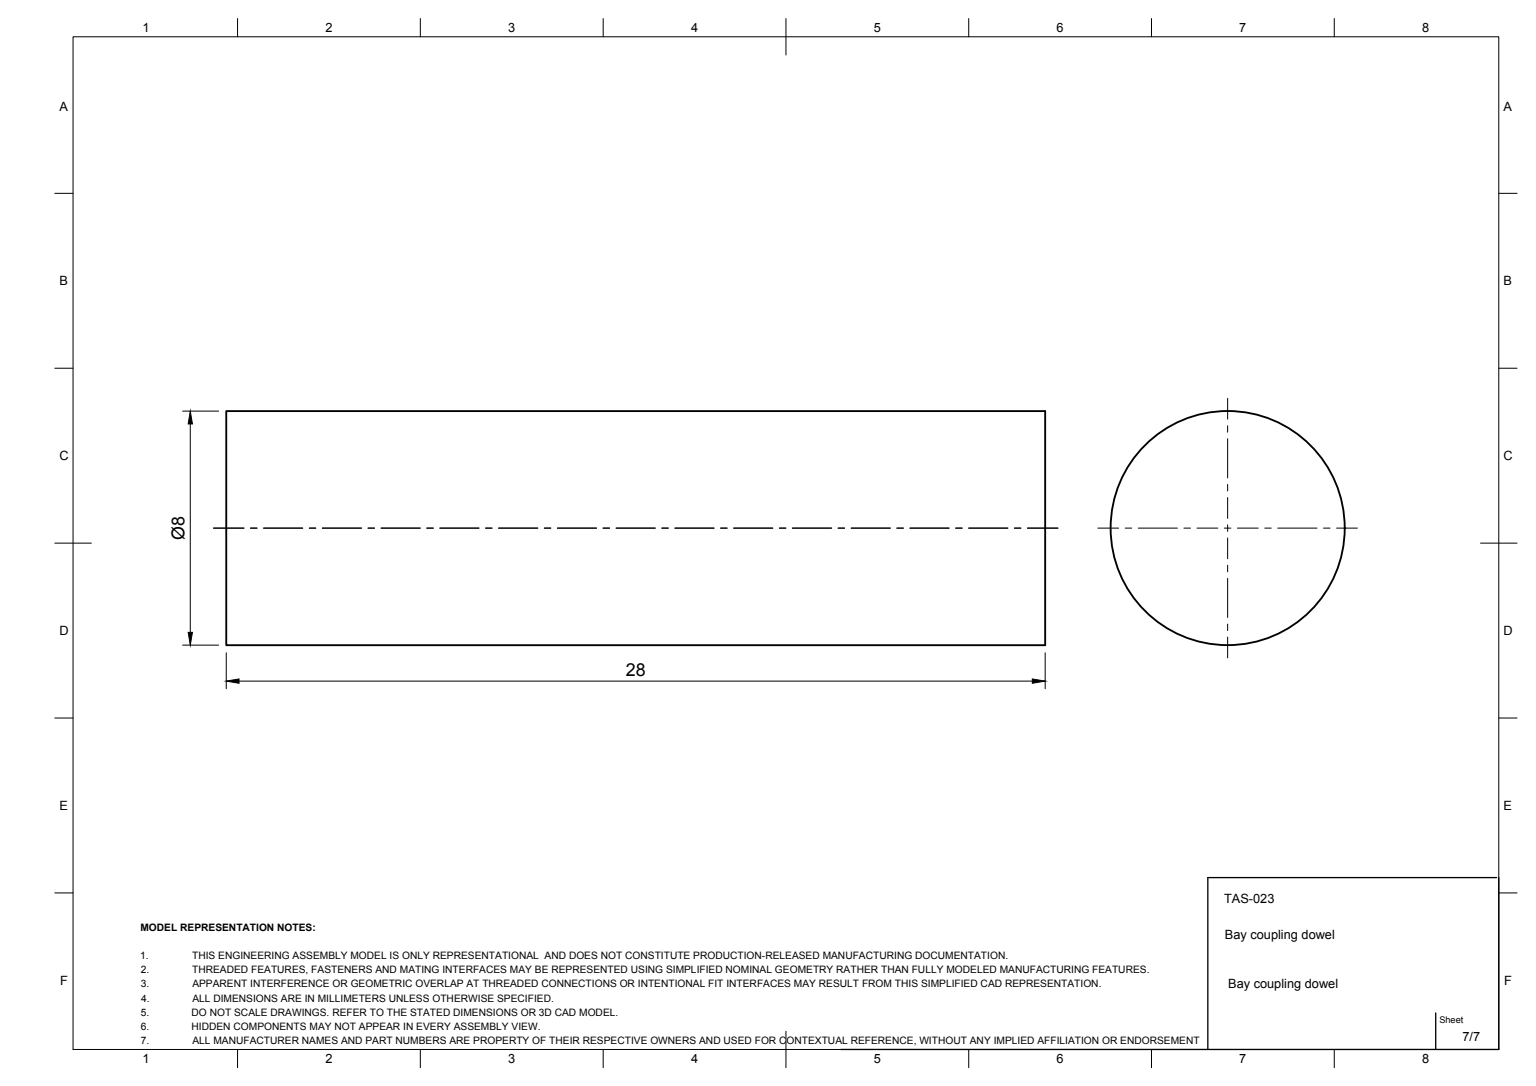
ISO-10303-21;
HEADER;
/* Generated by software containing ST-Developer
 * from STEP Tools, Inc. (www.steptools.com) 
 */

FILE_DESCRIPTION(
/* description */ (''),
/* implementation_level */ '2;1');

FILE_NAME(
/* name */ 'Bay coupling dowel.step',
/* time_stamp */ '2026-11-15T17:51:54-08:00',
/* author */ (''),
/* organization */ (''),
/* preprocessor_version */ 'ST-DEVELOPER v20.2',
/* originating_system */ 'Autodesk Translation Framework v15.17.0.0',
/* authorisation */ '');

FILE_SCHEMA (('AUTOMOTIVE_DESIGN { 1 0 10303 214 3 1 1 }'));
ENDSEC;

DATA;
#10=MECHANICAL_DESIGN_GEOMETRIC_PRESENTATION_REPRESENTATION('',(#121),#2860);
#111=SHAPE_REPRESENTATION_RELATIONSHIP('SRR','None',#2906,#116);
#116=ADVANCED_BREP_SHAPE_REPRESENTATION('',(#126),#2859);
#121=STYLED_ITEM('',(#2940),#126);
#126=MANIFOLD_SOLID_BREP('Body1',#1718);
#211=PLANE('',#1876);
#212=PLANE('',#1877);
#297=FACE_OUTER_BOUND('',#388,.T.);
#298=FACE_OUTER_BOUND('',#389,.T.);
#299=FACE_OUTER_BOUND('',#390,.T.);
#388=EDGE_LOOP('',(#1616,#1617,#1618,#1619));
#389=EDGE_LOOP('',(#1620));
#390=EDGE_LOOP('',(#1621));
#599=LINE('',#2819,#808);
#808=VECTOR('',#2310,0.4);
#817=CIRCLE('',#1874,0.4);
#818=CIRCLE('',#1875,0.4);
#963=VERTEX_POINT('',#2816);
#964=VERTEX_POINT('',#2818);
#1181=EDGE_CURVE('',#963,#963,#817,.T.);
#1182=EDGE_CURVE('',#963,#964,#599,.T.);
#1183=EDGE_CURVE('',#964,#964,#818,.T.);
#1616=ORIENTED_EDGE('',*,*,#1181,.F.);
#1617=ORIENTED_EDGE('',*,*,#1182,.T.);
#1618=ORIENTED_EDGE('',*,*,#1183,.T.);
#1619=ORIENTED_EDGE('',*,*,#1182,.F.);
#1620=ORIENTED_EDGE('',*,*,#1181,.T.);
#1621=ORIENTED_EDGE('',*,*,#1183,.F.);
#1626=CYLINDRICAL_SURFACE('',#1873,0.4);
#1711=ADVANCED_FACE('',(#297),#1626,.T.);
#1712=ADVANCED_FACE('',(#298),#211,.T.);
#1713=ADVANCED_FACE('',(#299),#212,.F.);
#1718=CLOSED_SHELL('',(#1711,#1712,#1713));
#1872=AXIS2_PLACEMENT_3D('',#2814,#2304,#2305);
#1873=AXIS2_PLACEMENT_3D('',#2815,#2306,#2307);
#1874=AXIS2_PLACEMENT_3D('',#2817,#2308,#2309);
#1875=AXIS2_PLACEMENT_3D('',#2820,#2311,#2312);
#1876=AXIS2_PLACEMENT_3D('',#2821,#2313,#2314);
#1877=AXIS2_PLACEMENT_3D('',#2822,#2315,#2316);
#2304=DIRECTION('axis',(0.,0.,1.));
#2305=DIRECTION('refdir',(1.,0.,0.));
#2306=DIRECTION('center_axis',(0.,0.,1.));
#2307=DIRECTION('ref_axis',(1.,0.,0.));
#2308=DIRECTION('center_axis',(0.,0.,1.));
#2309=DIRECTION('ref_axis',(1.,0.,0.));
#2310=DIRECTION('',(0.,0.,-1.));
#2311=DIRECTION('center_axis',(0.,0.,1.));
#2312=DIRECTION('ref_axis',(1.,0.,0.));
#2313=DIRECTION('center_axis',(0.,0.,1.));
#2314=DIRECTION('ref_axis',(1.,0.,0.));
#2315=DIRECTION('center_axis',(0.,0.,1.));
#2316=DIRECTION('ref_axis',(1.,0.,0.));
#2814=CARTESIAN_POINT('',(0.,0.,0.));
#2815=CARTESIAN_POINT('Origin',(0.,0.,0.));
#2816=CARTESIAN_POINT('',(-0.4,-4.89858719658941E-17,2.8));
#2817=CARTESIAN_POINT('Origin',(0.,0.,2.8));
#2818=CARTESIAN_POINT('',(-0.4,-4.89858719658941E-17,0.));
#2819=CARTESIAN_POINT('',(-0.4,-4.89858719658941E-17,0.));
#2820=CARTESIAN_POINT('Origin',(0.,0.,0.));
#2821=CARTESIAN_POINT('Origin',(0.,0.,2.8));
#2822=CARTESIAN_POINT('Origin',(0.,0.,0.));
#2852=UNCERTAINTY_MEASURE_WITH_UNIT(LENGTH_MEASURE(0.001),#2861,
'DISTANCE_ACCURACY_VALUE',
'Maximum model space distance between geometric entities at asserted c
onnectivities');
#2853=UNCERTAINTY_MEASURE_WITH_UNIT(LENGTH_MEASURE(0.001),#2861,
'DISTANCE_ACCURACY_VALUE',
'Maximum model space distance between geometric entities at asserted c
onnectivities');
#2859=(
GEOMETRIC_REPRESENTATION_CONTEXT(3)
GLOBAL_UNCERTAINTY_ASSIGNED_CONTEXT((#2852))
GLOBAL_UNIT_ASSIGNED_CONTEXT((#2861,#2863,#2864))
REPRESENTATION_CONTEXT('','3D')
);
#2860=(
GEOMETRIC_REPRESENTATION_CONTEXT(3)
GLOBAL_UNCERTAINTY_ASSIGNED_CONTEXT((#2853))
GLOBAL_UNIT_ASSIGNED_CONTEXT((#2861,#2863,#2864))
REPRESENTATION_CONTEXT('','3D')
);
#2861=(
LENGTH_UNIT()
NAMED_UNIT(*)
SI_UNIT(.CENTI.,.METRE.)
);
#2863=(
NAMED_UNIT(*)
PLANE_ANGLE_UNIT()
SI_UNIT($,.RADIAN.)
);
#2864=(
NAMED_UNIT(*)
SI_UNIT($,.STERADIAN.)
SOLID_ANGLE_UNIT()
);
#2870=SHAPE_DEFINITION_REPRESENTATION(#2876,#2906);
#2876=PRODUCT_DEFINITION_SHAPE('',$,#2913);
#2906=SHAPE_REPRESENTATION('',(#1872),#2859);
#2907=PRODUCT_DEFINITION_CONTEXT('part definition',#2927,'design');
#2913=PRODUCT_DEFINITION('Bay coupling dowel','Bay coupling dowel',#2919,
#2907);
#2919=PRODUCT_DEFINITION_FORMATION('',$,#2934);
#2927=APPLICATION_CONTEXT(
'Core Data for Automotive Mechanical Design Process');
#2928=PRODUCT_CONTEXT('part definition',#2927,'mechanical');
#2934=PRODUCT('Bay coupling dowel','Bay coupling dowel',$,(#2928));
#2940=PRESENTATION_STYLE_ASSIGNMENT((#2946));
#2946=SURFACE_STYLE_USAGE(.BOTH.,#2952);
#2952=SURFACE_SIDE_STYLE('',(#2958));
#2958=SURFACE_STYLE_FILL_AREA(#2964);
#2964=FILL_AREA_STYLE('Bay coupling dowel finish',(#2970));
#2970=FILL_AREA_STYLE_COLOUR('Bay coupling dowel finish',#2976);
#2976=COLOUR_RGB('Bay coupling dowel finish',0.43921568627451,0.47843137254902,
0.52156862745098);
ENDSEC;
END-ISO-10303-21;
